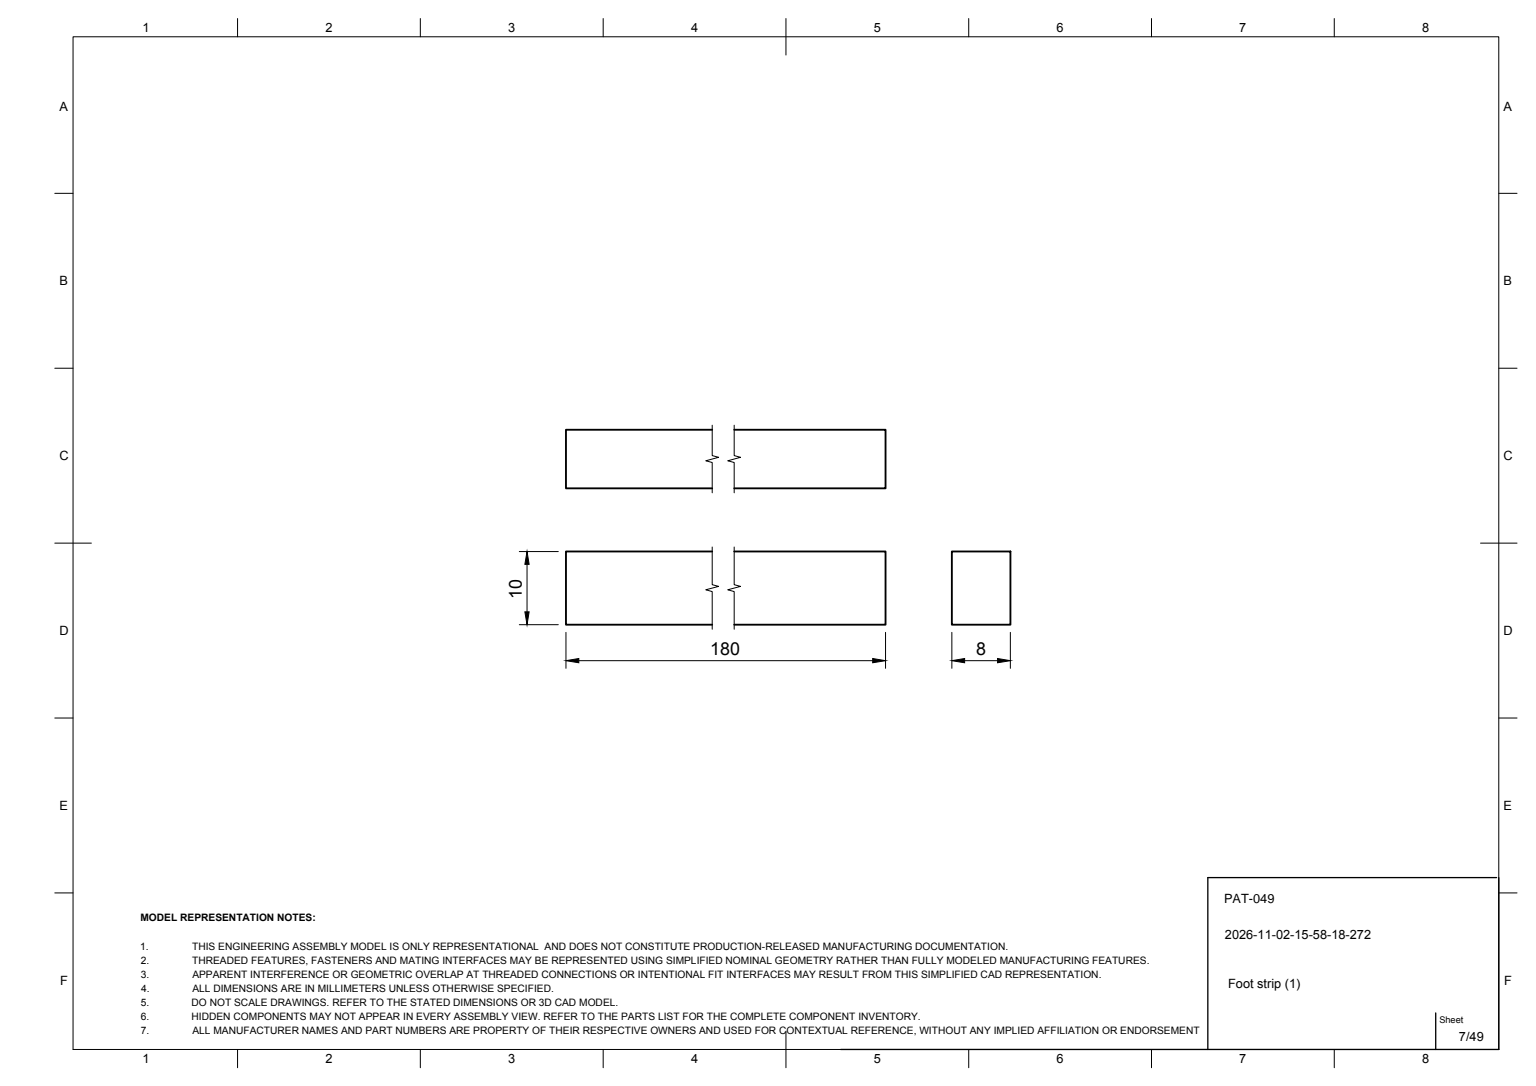
ISO-10303-21;
HEADER;
/* Generated by software containing ST-Developer
 * from STEP Tools, Inc. (www.steptools.com) 
 */

FILE_DESCRIPTION(
/* description */ ('Hand drill press frame (manual)'),
/* implementation_level */ '2;1');

FILE_NAME(
/* name */ 'Foot strip (1).step',
/* time_stamp */ '2026-10-28T03:25:28-07:00',
/* author */ (''),
/* organization */ (''),
/* preprocessor_version */ 'ST-DEVELOPER v20.2',
/* originating_system */ 'Autodesk Translation Framework v15.17.0.0',
/* authorisation */ '');

FILE_SCHEMA (('AUTOMOTIVE_DESIGN { 1 0 10303 214 3 1 1 }'));
ENDSEC;

DATA;
#10=MECHANICAL_DESIGN_GEOMETRIC_PRESENTATION_REPRESENTATION('',(#621),#33299);
#531=SHAPE_REPRESENTATION_RELATIONSHIP('SRR','None',#33490,#576);
#576=ADVANCED_BREP_SHAPE_REPRESENTATION('',(#673),#33252);
#621=STYLED_ITEM('',(#33800),#673);
#673=MANIFOLD_SOLID_BREP('Body1',#12639);
#899=PLANE('',#13223);
#900=PLANE('',#13224);
#901=PLANE('',#13225);
#902=PLANE('',#13226);
#903=PLANE('',#13227);
#904=PLANE('',#13228);
#1357=FACE_OUTER_BOUND('',#2058,.T.);
#1358=FACE_OUTER_BOUND('',#2059,.T.);
#1359=FACE_OUTER_BOUND('',#2060,.T.);
#1360=FACE_OUTER_BOUND('',#2061,.T.);
#1361=FACE_OUTER_BOUND('',#2062,.T.);
#1362=FACE_OUTER_BOUND('',#2063,.T.);
#2058=EDGE_LOOP('',(#8505,#8506,#8507,#8508));
#2059=EDGE_LOOP('',(#8509,#8510,#8511,#8512));
#2060=EDGE_LOOP('',(#8513,#8514,#8515,#8516));
#2061=EDGE_LOOP('',(#8517,#8518,#8519,#8520));
#2062=EDGE_LOOP('',(#8521,#8522,#8523,#8524));
#2063=EDGE_LOOP('',(#8525,#8526,#8527,#8528));
#2914=LINE('',#17986,#4079);
#2915=LINE('',#17988,#4080);
#2916=LINE('',#17990,#4081);
#2917=LINE('',#17991,#4082);
#2918=LINE('',#17994,#4083);
#2919=LINE('',#17996,#4084);
#2920=LINE('',#17997,#4085);
#2921=LINE('',#18000,#4086);
#2922=LINE('',#18002,#4087);
#2923=LINE('',#18003,#4088);
#2924=LINE('',#18005,#4089);
#2925=LINE('',#18006,#4090);
#4079=VECTOR('',#14469,1.);
#4080=VECTOR('',#14470,1.);
#4081=VECTOR('',#14471,1.);
#4082=VECTOR('',#14472,1.);
#4083=VECTOR('',#14475,1.);
#4084=VECTOR('',#14476,1.);
#4085=VECTOR('',#14477,1.);
#4086=VECTOR('',#14480,1.);
#4087=VECTOR('',#14481,1.);
#4088=VECTOR('',#14482,1.);
#4089=VECTOR('',#14485,1.);
#4090=VECTOR('',#14486,1.);
#5641=VERTEX_POINT('',#17984);
#5642=VERTEX_POINT('',#17985);
#5643=VERTEX_POINT('',#17987);
#5644=VERTEX_POINT('',#17989);
#5645=VERTEX_POINT('',#17993);
#5646=VERTEX_POINT('',#17995);
#5647=VERTEX_POINT('',#17999);
#5648=VERTEX_POINT('',#18001);
#6781=EDGE_CURVE('',#5641,#5642,#2914,.T.);
#6782=EDGE_CURVE('',#5642,#5643,#2915,.T.);
#6783=EDGE_CURVE('',#5644,#5643,#2916,.T.);
#6784=EDGE_CURVE('',#5641,#5644,#2917,.T.);
#6785=EDGE_CURVE('',#5645,#5641,#2918,.T.);
#6786=EDGE_CURVE('',#5646,#5644,#2919,.T.);
#6787=EDGE_CURVE('',#5645,#5646,#2920,.T.);
#6788=EDGE_CURVE('',#5647,#5645,#2921,.T.);
#6789=EDGE_CURVE('',#5648,#5646,#2922,.T.);
#6790=EDGE_CURVE('',#5647,#5648,#2923,.T.);
#6791=EDGE_CURVE('',#5642,#5647,#2924,.T.);
#6792=EDGE_CURVE('',#5643,#5648,#2925,.T.);
#8505=ORIENTED_EDGE('',*,*,#6781,.T.);
#8506=ORIENTED_EDGE('',*,*,#6782,.T.);
#8507=ORIENTED_EDGE('',*,*,#6783,.F.);
#8508=ORIENTED_EDGE('',*,*,#6784,.F.);
#8509=ORIENTED_EDGE('',*,*,#6785,.T.);
#8510=ORIENTED_EDGE('',*,*,#6784,.T.);
#8511=ORIENTED_EDGE('',*,*,#6786,.F.);
#8512=ORIENTED_EDGE('',*,*,#6787,.F.);
#8513=ORIENTED_EDGE('',*,*,#6788,.T.);
#8514=ORIENTED_EDGE('',*,*,#6787,.T.);
#8515=ORIENTED_EDGE('',*,*,#6789,.F.);
#8516=ORIENTED_EDGE('',*,*,#6790,.F.);
#8517=ORIENTED_EDGE('',*,*,#6791,.T.);
#8518=ORIENTED_EDGE('',*,*,#6790,.T.);
#8519=ORIENTED_EDGE('',*,*,#6792,.F.);
#8520=ORIENTED_EDGE('',*,*,#6782,.F.);
#8521=ORIENTED_EDGE('',*,*,#6792,.T.);
#8522=ORIENTED_EDGE('',*,*,#6789,.T.);
#8523=ORIENTED_EDGE('',*,*,#6786,.T.);
#8524=ORIENTED_EDGE('',*,*,#6783,.T.);
#8525=ORIENTED_EDGE('',*,*,#6791,.F.);
#8526=ORIENTED_EDGE('',*,*,#6781,.F.);
#8527=ORIENTED_EDGE('',*,*,#6785,.F.);
#8528=ORIENTED_EDGE('',*,*,#6788,.F.);
#11966=ADVANCED_FACE('',(#1357),#899,.T.);
#11967=ADVANCED_FACE('',(#1358),#900,.T.);
#11968=ADVANCED_FACE('',(#1359),#901,.T.);
#11969=ADVANCED_FACE('',(#1360),#902,.T.);
#11970=ADVANCED_FACE('',(#1361),#903,.T.);
#11971=ADVANCED_FACE('',(#1362),#904,.F.);
#12639=CLOSED_SHELL('',(#11966,#11967,#11968,#11969,#11970,#11971));
#13222=AXIS2_PLACEMENT_3D('',#17982,#14465,#14466);
#13223=AXIS2_PLACEMENT_3D('',#17983,#14467,#14468);
#13224=AXIS2_PLACEMENT_3D('',#17992,#14473,#14474);
#13225=AXIS2_PLACEMENT_3D('',#17998,#14478,#14479);
#13226=AXIS2_PLACEMENT_3D('',#18004,#14483,#14484);
#13227=AXIS2_PLACEMENT_3D('',#18007,#14487,#14488);
#13228=AXIS2_PLACEMENT_3D('',#18008,#14489,#14490);
#14465=DIRECTION('axis',(0.,0.,1.));
#14466=DIRECTION('refdir',(1.,0.,0.));
#14467=DIRECTION('center_axis',(0.,1.,0.));
#14468=DIRECTION('ref_axis',(-1.,0.,0.));
#14469=DIRECTION('',(-1.,0.,0.));
#14470=DIRECTION('',(0.,0.,1.));
#14471=DIRECTION('',(-1.,0.,0.));
#14472=DIRECTION('',(0.,0.,1.));
#14473=DIRECTION('center_axis',(1.,0.,0.));
#14474=DIRECTION('ref_axis',(0.,1.,0.));
#14475=DIRECTION('',(0.,1.,0.));
#14476=DIRECTION('',(0.,1.,0.));
#14477=DIRECTION('',(0.,0.,1.));
#14478=DIRECTION('center_axis',(0.,-1.,0.));
#14479=DIRECTION('ref_axis',(1.,0.,0.));
#14480=DIRECTION('',(1.,0.,0.));
#14481=DIRECTION('',(1.,0.,0.));
#14482=DIRECTION('',(0.,0.,1.));
#14483=DIRECTION('center_axis',(-1.,0.,0.));
#14484=DIRECTION('ref_axis',(0.,-1.,0.));
#14485=DIRECTION('',(0.,-1.,0.));
#14486=DIRECTION('',(0.,-1.,0.));
#14487=DIRECTION('center_axis',(0.,0.,1.));
#14488=DIRECTION('ref_axis',(1.,0.,0.));
#14489=DIRECTION('center_axis',(0.,0.,1.));
#14490=DIRECTION('ref_axis',(1.,0.,0.));
#17982=CARTESIAN_POINT('',(0.,0.,0.));
#17983=CARTESIAN_POINT('Origin',(10.,9.,-0.8));
#17984=CARTESIAN_POINT('',(10.,9.,-0.8));
#17985=CARTESIAN_POINT('',(9.,9.,-0.8));
#17986=CARTESIAN_POINT('',(10.,9.,-0.8));
#17987=CARTESIAN_POINT('',(9.,9.,0.));
#17988=CARTESIAN_POINT('',(9.,9.,-0.8));
#17989=CARTESIAN_POINT('',(10.,9.,0.));
#17990=CARTESIAN_POINT('',(10.,9.,0.));
#17991=CARTESIAN_POINT('',(10.,9.,-0.8));
#17992=CARTESIAN_POINT('Origin',(10.,-9.,-0.8));
#17993=CARTESIAN_POINT('',(10.,-9.,-0.8));
#17994=CARTESIAN_POINT('',(10.,-9.,-0.8));
#17995=CARTESIAN_POINT('',(10.,-9.,0.));
#17996=CARTESIAN_POINT('',(10.,-9.,0.));
#17997=CARTESIAN_POINT('',(10.,-9.,-0.8));
#17998=CARTESIAN_POINT('Origin',(9.,-9.,-0.8));
#17999=CARTESIAN_POINT('',(9.,-9.,-0.8));
#18000=CARTESIAN_POINT('',(9.,-9.,-0.8));
#18001=CARTESIAN_POINT('',(9.,-9.,0.));
#18002=CARTESIAN_POINT('',(9.,-9.,0.));
#18003=CARTESIAN_POINT('',(9.,-9.,-0.8));
#18004=CARTESIAN_POINT('Origin',(9.,9.,-0.8));
#18005=CARTESIAN_POINT('',(9.,9.,-0.8));
#18006=CARTESIAN_POINT('',(9.,9.,0.));
#18007=CARTESIAN_POINT('Origin',(9.5,0.,0.));
#18008=CARTESIAN_POINT('Origin',(9.5,0.,-0.8));
#33200=UNCERTAINTY_MEASURE_WITH_UNIT(LENGTH_MEASURE(0.001),#33300,
'DISTANCE_ACCURACY_VALUE',
'Maximum model space distance between geometric entities at asserted c
onnectivities');
#33247=UNCERTAINTY_MEASURE_WITH_UNIT(LENGTH_MEASURE(0.001),#33300,
'DISTANCE_ACCURACY_VALUE',
'Maximum model space distance between geometric entities at asserted c
onnectivities');
#33252=(
GEOMETRIC_REPRESENTATION_CONTEXT(3)
GLOBAL_UNCERTAINTY_ASSIGNED_CONTEXT((#33200))
GLOBAL_UNIT_ASSIGNED_CONTEXT((#33300,#33302,#33303))
REPRESENTATION_CONTEXT('','3D')
);
#33299=(
GEOMETRIC_REPRESENTATION_CONTEXT(3)
GLOBAL_UNCERTAINTY_ASSIGNED_CONTEXT((#33247))
GLOBAL_UNIT_ASSIGNED_CONTEXT((#33300,#33302,#33303))
REPRESENTATION_CONTEXT('','3D')
);
#33300=(
LENGTH_UNIT()
NAMED_UNIT(*)
SI_UNIT(.CENTI.,.METRE.)
);
#33302=(
NAMED_UNIT(*)
PLANE_ANGLE_UNIT()
SI_UNIT($,.RADIAN.)
);
#33303=(
NAMED_UNIT(*)
SI_UNIT($,.STERADIAN.)
SOLID_ANGLE_UNIT()
);
#33308=SHAPE_DEFINITION_REPRESENTATION(#33359,#33490);
#33359=PRODUCT_DEFINITION_SHAPE('',$,#33542);
#33490=SHAPE_REPRESENTATION('',(#13222),#33252);
#33537=PRODUCT_DEFINITION_CONTEXT('part definition',#33692,'design');
#33542=PRODUCT_DEFINITION('Foot strip (1)','Foot strip (1)',#33593,#33537);
#33593=PRODUCT_DEFINITION_FORMATION('',$,#33698);
#33692=APPLICATION_CONTEXT(
'Core Data for Automotive Mechanical Design Process');
#33693=PRODUCT_CONTEXT('part definition',#33692,'mechanical');
#33698=PRODUCT('Foot strip (1)','Foot strip (1)','Foot strip (1)',(#33693));
#33794=COLOUR_RGB('Light Blue',0.38,0.62,0.78);
#33795=FILL_AREA_STYLE_COLOUR('',#33794);
#33796=FILL_AREA_STYLE('',(#33795));
#33797=SURFACE_STYLE_FILL_AREA(#33796);
#33798=SURFACE_SIDE_STYLE('',(#33797));
#33799=SURFACE_STYLE_USAGE(.BOTH.,#33798);
#33800=PRESENTATION_STYLE_ASSIGNMENT((#33799));
ENDSEC;
END-ISO-10303-21;
